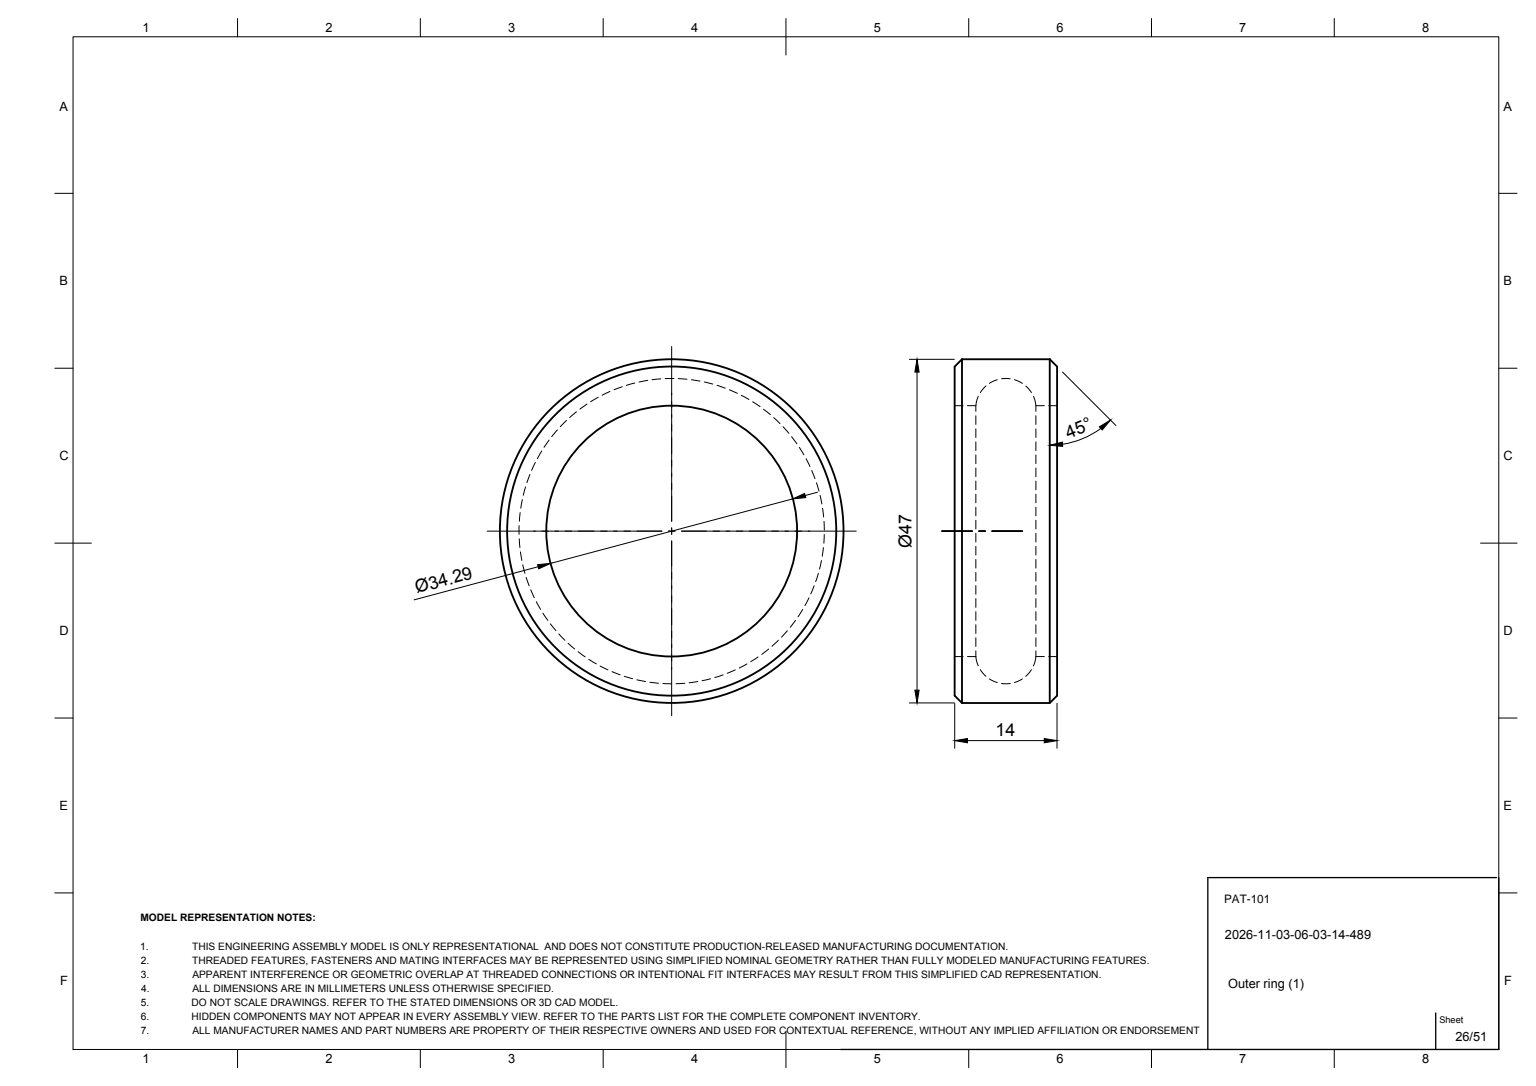
ISO-10303-21;
HEADER;
/* Generated by software containing ST-Developer
 * from STEP Tools, Inc. (www.steptools.com) 
 */

FILE_DESCRIPTION(
/* description */ ('Spur gear reduction stage 2-1 on bearing plates'),
/* implementation_level */ '2;1');

FILE_NAME(
/* name */ 'Outer ring (1).step',
/* time_stamp */ '2026-10-28T03:22:07-07:00',
/* author */ (''),
/* organization */ (''),
/* preprocessor_version */ 'ST-DEVELOPER v20.2',
/* originating_system */ 'Autodesk Translation Framework v15.17.0.0',
/* authorisation */ '');

FILE_SCHEMA (('AUTOMOTIVE_DESIGN { 1 0 10303 214 3 1 1 }'));
ENDSEC;

DATA;
#10=MECHANICAL_DESIGN_GEOMETRIC_PRESENTATION_REPRESENTATION('',(#973),#53909);
#828=TOROIDAL_SURFACE('',#12303,1.675,0.412776);
#846=CONICAL_SURFACE('',#12314,2.3,0.785398163397449);
#847=CONICAL_SURFACE('',#12318,2.3,0.785398163397449);
#880=SHAPE_REPRESENTATION_RELATIONSHIP('SRR','None',#54109,#923);
#923=ADVANCED_BREP_SHAPE_REPRESENTATION('',(#1029),#53883);
#973=STYLED_ITEM('',(#54397),#1029);
#1029=MANIFOLD_SOLID_BREP('Body1',#11299);
#1189=FACE_BOUND('',#2503,.T.);
#1190=FACE_BOUND('',#2508,.T.);
#1332=PLANE('',#12311);
#1333=PLANE('',#12320);
#1723=FACE_OUTER_BOUND('',#2500,.T.);
#1724=FACE_OUTER_BOUND('',#2501,.T.);
#1725=FACE_OUTER_BOUND('',#2502,.T.);
#1726=FACE_OUTER_BOUND('',#2504,.T.);
#1727=FACE_OUTER_BOUND('',#2505,.T.);
#1728=FACE_OUTER_BOUND('',#2506,.T.);
#1729=FACE_OUTER_BOUND('',#2507,.T.);
#1730=FACE_OUTER_BOUND('',#2509,.T.);
#2500=EDGE_LOOP('',(#8238,#8239,#8240,#8241,#8242,#8243));
#2501=EDGE_LOOP('',(#8244,#8245,#8246,#8247,#8248));
#2502=EDGE_LOOP('',(#8249));
#2503=EDGE_LOOP('',(#8250));
#2504=EDGE_LOOP('',(#8251,#8252,#8253,#8254));
#2505=EDGE_LOOP('',(#8255,#8256,#8257,#8258));
#2506=EDGE_LOOP('',(#8259,#8260,#8261,#8262));
#2507=EDGE_LOOP('',(#8263));
#2508=EDGE_LOOP('',(#8264));
#2509=EDGE_LOOP('',(#8265,#8266,#8267,#8268,#8269));
#3158=LINE('',#17274,#3799);
#3159=LINE('',#17283,#3800);
#3160=LINE('',#17287,#3801);
#3161=LINE('',#17291,#3802);
#3162=LINE('',#17294,#3803);
#3799=VECTOR('',#14173,1.71469);
#3800=VECTOR('',#14184,2.3);
#3801=VECTOR('',#14189,2.35);
#3802=VECTOR('',#14194,2.3);
#3803=VECTOR('',#14199,1.71469);
#4507=CIRCLE('',#12304,1.71469);
#4508=CIRCLE('',#12305,1.71469);
#4509=CIRCLE('',#12306,0.412776);
#4510=CIRCLE('',#12307,1.71469);
#4511=CIRCLE('',#12308,1.71469);
#4512=CIRCLE('',#12310,1.71469);
#4513=CIRCLE('',#12312,2.25);
#4514=CIRCLE('',#12313,1.71469);
#4515=CIRCLE('',#12315,2.35);
#4516=CIRCLE('',#12317,2.35);
#4517=CIRCLE('',#12319,2.25);
#5084=VERTEX_POINT('',#17262);
#5085=VERTEX_POINT('',#17263);
#5086=VERTEX_POINT('',#17266);
#5087=VERTEX_POINT('',#17268);
#5088=VERTEX_POINT('',#17272);
#5089=VERTEX_POINT('',#17276);
#5090=VERTEX_POINT('',#17278);
#5091=VERTEX_POINT('',#17281);
#5092=VERTEX_POINT('',#17285);
#5093=VERTEX_POINT('',#17289);
#6261=EDGE_CURVE('',#5084,#5085,#4507,.T.);
#6262=EDGE_CURVE('',#5085,#5084,#4508,.T.);
#6263=EDGE_CURVE('',#5085,#5086,#4509,.T.);
#6264=EDGE_CURVE('',#5087,#5086,#4510,.T.);
#6265=EDGE_CURVE('',#5086,#5087,#4511,.T.);
#6266=EDGE_CURVE('',#5088,#5088,#4512,.T.);
#6267=EDGE_CURVE('',#5088,#5087,#3158,.T.);
#6268=EDGE_CURVE('',#5089,#5089,#4513,.T.);
#6269=EDGE_CURVE('',#5090,#5090,#4514,.T.);
#6270=EDGE_CURVE('',#5091,#5091,#4515,.T.);
#6271=EDGE_CURVE('',#5091,#5089,#3159,.T.);
#6272=EDGE_CURVE('',#5092,#5092,#4516,.T.);
#6273=EDGE_CURVE('',#5092,#5091,#3160,.T.);
#6274=EDGE_CURVE('',#5093,#5093,#4517,.T.);
#6275=EDGE_CURVE('',#5093,#5092,#3161,.T.);
#6276=EDGE_CURVE('',#5084,#5090,#3162,.T.);
#8238=ORIENTED_EDGE('',*,*,#6261,.F.);
#8239=ORIENTED_EDGE('',*,*,#6262,.F.);
#8240=ORIENTED_EDGE('',*,*,#6263,.T.);
#8241=ORIENTED_EDGE('',*,*,#6264,.F.);
#8242=ORIENTED_EDGE('',*,*,#6265,.F.);
#8243=ORIENTED_EDGE('',*,*,#6263,.F.);
#8244=ORIENTED_EDGE('',*,*,#6266,.T.);
#8245=ORIENTED_EDGE('',*,*,#6267,.T.);
#8246=ORIENTED_EDGE('',*,*,#6264,.T.);
#8247=ORIENTED_EDGE('',*,*,#6265,.T.);
#8248=ORIENTED_EDGE('',*,*,#6267,.F.);
#8249=ORIENTED_EDGE('',*,*,#6268,.F.);
#8250=ORIENTED_EDGE('',*,*,#6269,.T.);
#8251=ORIENTED_EDGE('',*,*,#6270,.F.);
#8252=ORIENTED_EDGE('',*,*,#6271,.T.);
#8253=ORIENTED_EDGE('',*,*,#6268,.T.);
#8254=ORIENTED_EDGE('',*,*,#6271,.F.);
#8255=ORIENTED_EDGE('',*,*,#6272,.F.);
#8256=ORIENTED_EDGE('',*,*,#6273,.T.);
#8257=ORIENTED_EDGE('',*,*,#6270,.T.);
#8258=ORIENTED_EDGE('',*,*,#6273,.F.);
#8259=ORIENTED_EDGE('',*,*,#6274,.F.);
#8260=ORIENTED_EDGE('',*,*,#6275,.T.);
#8261=ORIENTED_EDGE('',*,*,#6272,.T.);
#8262=ORIENTED_EDGE('',*,*,#6275,.F.);
#8263=ORIENTED_EDGE('',*,*,#6274,.T.);
#8264=ORIENTED_EDGE('',*,*,#6266,.F.);
#8265=ORIENTED_EDGE('',*,*,#6261,.T.);
#8266=ORIENTED_EDGE('',*,*,#6262,.T.);
#8267=ORIENTED_EDGE('',*,*,#6276,.T.);
#8268=ORIENTED_EDGE('',*,*,#6269,.F.);
#8269=ORIENTED_EDGE('',*,*,#6276,.F.);
#10515=CYLINDRICAL_SURFACE('',#12309,1.71469);
#10516=CYLINDRICAL_SURFACE('',#12316,2.35);
#10517=CYLINDRICAL_SURFACE('',#12321,1.71469);
#10843=ADVANCED_FACE('',(#1723),#828,.F.);
#10844=ADVANCED_FACE('',(#1724),#10515,.F.);
#10845=ADVANCED_FACE('',(#1725,#1189),#1332,.T.);
#10846=ADVANCED_FACE('',(#1726),#846,.T.);
#10847=ADVANCED_FACE('',(#1727),#10516,.T.);
#10848=ADVANCED_FACE('',(#1728),#847,.T.);
#10849=ADVANCED_FACE('',(#1729,#1190),#1333,.T.);
#10850=ADVANCED_FACE('',(#1730),#10517,.F.);
#11299=CLOSED_SHELL('',(#10843,#10844,#10845,#10846,#10847,#10848,#10849,
#10850));
#12302=AXIS2_PLACEMENT_3D('',#17260,#14155,#14156);
#12303=AXIS2_PLACEMENT_3D('',#17261,#14157,#14158);
#12304=AXIS2_PLACEMENT_3D('',#17264,#14159,#14160);
#12305=AXIS2_PLACEMENT_3D('',#17265,#14161,#14162);
#12306=AXIS2_PLACEMENT_3D('',#17267,#14163,#14164);
#12307=AXIS2_PLACEMENT_3D('',#17269,#14165,#14166);
#12308=AXIS2_PLACEMENT_3D('',#17270,#14167,#14168);
#12309=AXIS2_PLACEMENT_3D('',#17271,#14169,#14170);
#12310=AXIS2_PLACEMENT_3D('',#17273,#14171,#14172);
#12311=AXIS2_PLACEMENT_3D('',#17275,#14174,#14175);
#12312=AXIS2_PLACEMENT_3D('',#17277,#14176,#14177);
#12313=AXIS2_PLACEMENT_3D('',#17279,#14178,#14179);
#12314=AXIS2_PLACEMENT_3D('',#17280,#14180,#14181);
#12315=AXIS2_PLACEMENT_3D('',#17282,#14182,#14183);
#12316=AXIS2_PLACEMENT_3D('',#17284,#14185,#14186);
#12317=AXIS2_PLACEMENT_3D('',#17286,#14187,#14188);
#12318=AXIS2_PLACEMENT_3D('',#17288,#14190,#14191);
#12319=AXIS2_PLACEMENT_3D('',#17290,#14192,#14193);
#12320=AXIS2_PLACEMENT_3D('',#17292,#14195,#14196);
#12321=AXIS2_PLACEMENT_3D('',#17293,#14197,#14198);
#14155=DIRECTION('axis',(0.,0.,1.));
#14156=DIRECTION('refdir',(1.,0.,0.));
#14157=DIRECTION('center_axis',(0.,-1.,0.));
#14158=DIRECTION('ref_axis',(0.,0.,-1.));
#14159=DIRECTION('center_axis',(0.,-1.,0.));
#14160=DIRECTION('ref_axis',(1.,0.,0.));
#14161=DIRECTION('center_axis',(0.,-1.,0.));
#14162=DIRECTION('ref_axis',(1.,0.,0.));
#14163=DIRECTION('center_axis',(1.,0.,1.22464679914735E-16));
#14164=DIRECTION('ref_axis',(-1.22464679914735E-16,0.,1.));
#14165=DIRECTION('center_axis',(0.,1.,0.));
#14166=DIRECTION('ref_axis',(1.,0.,0.));
#14167=DIRECTION('center_axis',(0.,1.,0.));
#14168=DIRECTION('ref_axis',(1.,0.,0.));
#14169=DIRECTION('center_axis',(0.,-1.,0.));
#14170=DIRECTION('ref_axis',(1.,0.,0.));
#14171=DIRECTION('center_axis',(0.,-1.,0.));
#14172=DIRECTION('ref_axis',(1.,0.,0.));
#14173=DIRECTION('',(0.,1.,0.));
#14174=DIRECTION('center_axis',(0.,1.,0.));
#14175=DIRECTION('ref_axis',(0.,0.,1.));
#14176=DIRECTION('center_axis',(0.,-1.,0.));
#14177=DIRECTION('ref_axis',(1.,0.,0.));
#14178=DIRECTION('center_axis',(0.,-1.,0.));
#14179=DIRECTION('ref_axis',(1.,0.,0.));
#14180=DIRECTION('center_axis',(0.,-1.,0.));
#14181=DIRECTION('ref_axis',(1.,0.,0.));
#14182=DIRECTION('center_axis',(0.,-1.,0.));
#14183=DIRECTION('ref_axis',(1.,0.,0.));
#14184=DIRECTION('',(0.707106781186548,0.707106781186547,8.65956056235494E-17));
#14185=DIRECTION('center_axis',(0.,-1.,0.));
#14186=DIRECTION('ref_axis',(1.,0.,0.));
#14187=DIRECTION('center_axis',(0.,-1.,0.));
#14188=DIRECTION('ref_axis',(1.,0.,0.));
#14189=DIRECTION('',(0.,1.,0.));
#14190=DIRECTION('center_axis',(0.,1.,0.));
#14191=DIRECTION('ref_axis',(1.,0.,0.));
#14192=DIRECTION('center_axis',(0.,-1.,0.));
#14193=DIRECTION('ref_axis',(1.,0.,0.));
#14194=DIRECTION('',(-0.707106781186548,0.707106781186547,-8.65956056235494E-17));
#14195=DIRECTION('center_axis',(0.,-1.,0.));
#14196=DIRECTION('ref_axis',(0.,0.,-1.));
#14197=DIRECTION('center_axis',(0.,-1.,0.));
#14198=DIRECTION('ref_axis',(1.,0.,0.));
#14199=DIRECTION('',(0.,1.,0.));
#17260=CARTESIAN_POINT('',(0.,0.,0.));
#17261=CARTESIAN_POINT('Origin',(0.,0.,0.));
#17262=CARTESIAN_POINT('',(-1.71469,0.410863395882378,-2.09988962002998E-16));
#17263=CARTESIAN_POINT('',(-2.09988962002998E-16,0.410863395882378,1.71469));
#17264=CARTESIAN_POINT('Origin',(0.,0.410863395882378,0.));
#17265=CARTESIAN_POINT('Origin',(0.,0.410863395882378,0.));
#17266=CARTESIAN_POINT('',(-2.09988962002998E-16,-0.410863395882378,1.71469));
#17267=CARTESIAN_POINT('Origin',(-2.05128338857182E-16,0.,1.675));
#17268=CARTESIAN_POINT('',(-1.71469,-0.410863395882378,2.09988962002998E-16));
#17269=CARTESIAN_POINT('Origin',(0.,-0.410863395882378,0.));
#17270=CARTESIAN_POINT('Origin',(0.,-0.410863395882378,0.));
#17271=CARTESIAN_POINT('Origin',(0.,0.,0.));
#17272=CARTESIAN_POINT('',(-1.71469,-0.7,-2.09988962002998E-16));
#17273=CARTESIAN_POINT('Origin',(0.,-0.7,0.));
#17274=CARTESIAN_POINT('',(-1.71469,0.,-2.09988962002998E-16));
#17275=CARTESIAN_POINT('Origin',(2.25,0.7,0.));
#17276=CARTESIAN_POINT('',(-2.25,0.7,-2.75545529808154E-16));
#17277=CARTESIAN_POINT('Origin',(0.,0.7,0.));
#17278=CARTESIAN_POINT('',(-1.71469,0.7,-2.09988962002998E-16));
#17279=CARTESIAN_POINT('Origin',(0.,0.7,0.));
#17280=CARTESIAN_POINT('Origin',(0.,0.65,0.));
#17281=CARTESIAN_POINT('',(-2.35,0.6,-2.87791997799628E-16));
#17282=CARTESIAN_POINT('Origin',(0.,0.6,0.));
#17283=CARTESIAN_POINT('',(-2.3,0.65,-2.81668763803891E-16));
#17284=CARTESIAN_POINT('Origin',(0.,0.,0.));
#17285=CARTESIAN_POINT('',(-2.35,-0.6,-2.87791997799628E-16));
#17286=CARTESIAN_POINT('Origin',(0.,-0.6,0.));
#17287=CARTESIAN_POINT('',(-2.35,0.,-2.87791997799628E-16));
#17288=CARTESIAN_POINT('Origin',(0.,-0.65,0.));
#17289=CARTESIAN_POINT('',(-2.25,-0.7,-2.75545529808154E-16));
#17290=CARTESIAN_POINT('Origin',(0.,-0.7,0.));
#17291=CARTESIAN_POINT('',(-2.3,-0.65,-2.81668763803891E-16));
#17292=CARTESIAN_POINT('Origin',(1.71469,-0.7,0.));
#17293=CARTESIAN_POINT('Origin',(0.,0.,0.));
#17294=CARTESIAN_POINT('',(-1.71469,0.,-2.09988962002998E-16));
#53833=UNCERTAINTY_MEASURE_WITH_UNIT(LENGTH_MEASURE(0.001),#53910,
'DISTANCE_ACCURACY_VALUE',
'Maximum model space distance between geometric entities at asserted c
onnectivities');
#53859=UNCERTAINTY_MEASURE_WITH_UNIT(LENGTH_MEASURE(0.001),#53910,
'DISTANCE_ACCURACY_VALUE',
'Maximum model space distance between geometric entities at asserted c
onnectivities');
#53883=(
GEOMETRIC_REPRESENTATION_CONTEXT(3)
GLOBAL_UNCERTAINTY_ASSIGNED_CONTEXT((#53833))
GLOBAL_UNIT_ASSIGNED_CONTEXT((#53910,#53912,#53913))
REPRESENTATION_CONTEXT('','3D')
);
#53909=(
GEOMETRIC_REPRESENTATION_CONTEXT(3)
GLOBAL_UNCERTAINTY_ASSIGNED_CONTEXT((#53859))
GLOBAL_UNIT_ASSIGNED_CONTEXT((#53910,#53912,#53913))
REPRESENTATION_CONTEXT('','3D')
);
#53910=(
LENGTH_UNIT()
NAMED_UNIT(*)
SI_UNIT(.CENTI.,.METRE.)
);
#53912=(
NAMED_UNIT(*)
PLANE_ANGLE_UNIT()
SI_UNIT($,.RADIAN.)
);
#53913=(
NAMED_UNIT(*)
SI_UNIT($,.STERADIAN.)
SOLID_ANGLE_UNIT()
);
#53937=SHAPE_DEFINITION_REPRESENTATION(#53991,#54109);
#53991=PRODUCT_DEFINITION_SHAPE('',$,#54159);
#54109=SHAPE_REPRESENTATION('',(#12302),#53883);
#54135=PRODUCT_DEFINITION_CONTEXT('part definition',#54284,'design');
#54159=PRODUCT_DEFINITION('Outer ring (1)','Outer ring (1)',#54208,#54135);
#54208=PRODUCT_DEFINITION_FORMATION('',$,#54309);
#54284=APPLICATION_CONTEXT(
'Core Data for Automotive Mechanical Design Process');
#54285=PRODUCT_CONTEXT('part definition',#54284,'mechanical');
#54309=PRODUCT('Outer ring (1)','Outer ring (1)','Outer ring (1)',(#54285));
#54391=COLOUR_RGB('Grey',0.48,0.52,0.57);
#54392=FILL_AREA_STYLE_COLOUR('',#54391);
#54393=FILL_AREA_STYLE('',(#54392));
#54394=SURFACE_STYLE_FILL_AREA(#54393);
#54395=SURFACE_SIDE_STYLE('',(#54394));
#54396=SURFACE_STYLE_USAGE(.BOTH.,#54395);
#54397=PRESENTATION_STYLE_ASSIGNMENT((#54396));
ENDSEC;
END-ISO-10303-21;
